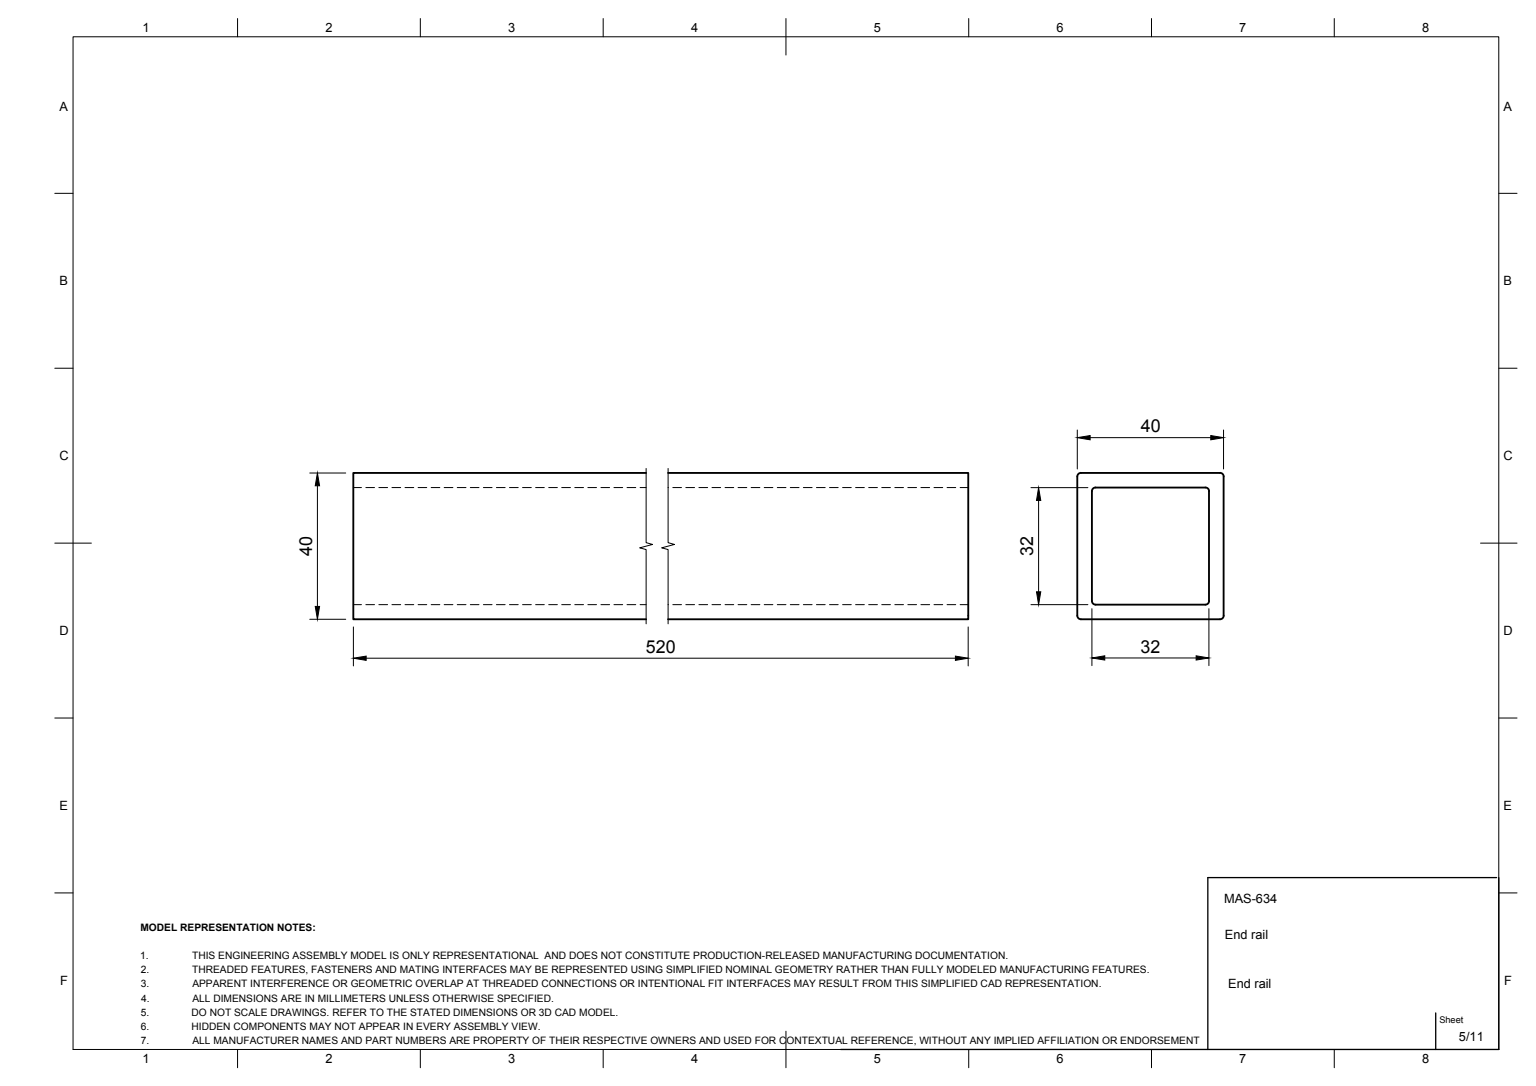
ISO-10303-21;
HEADER;
/* Generated by software containing ST-Developer
 * from STEP Tools, Inc. (www.steptools.com) 
 */

FILE_DESCRIPTION(
/* description */ ('Independent AHU equipment rack. Nominal800x600 frame on1000long40squa
re aluminum posts; two removable notched shelves; welded perimeter/cro
ss rails and rear gussets; two mounting channels; four isolation pads 
and anchor-ready feet. Imported native extrusion library retained and 
cut-length parameters customized per family. Shelf hardware uses model
ed M6 rivet nuts and screws. Weld design, floor anchors and load ratin
g require engineering selection.'),
/* implementation_level */ '2;1');

FILE_NAME(
/* name */ 'End rail.step',
/* time_stamp */ '2026-11-07T19:04:45-08:00',
/* author */ (''),
/* organization */ (''),
/* preprocessor_version */ 'ST-DEVELOPER v20.2',
/* originating_system */ 'Autodesk Translation Framework v15.17.0.0',
/* authorisation */ '');

FILE_SCHEMA (('AUTOMOTIVE_DESIGN { 1 0 10303 214 3 1 1 }'));
ENDSEC;

DATA;
#10=MECHANICAL_DESIGN_GEOMETRIC_PRESENTATION_REPRESENTATION('',(#337),#9777);
#315=SHAPE_REPRESENTATION_RELATIONSHIP('SRR','None',#9859,#326);
#326=ADVANCED_BREP_SHAPE_REPRESENTATION('',(#348),#9768);
#337=STYLED_ITEM('',(#9922),#348);
#348=MANIFOLD_SOLID_BREP('Aluminum square hollow profile',#3842);
#365=FACE_BOUND('',#749,.T.);
#366=FACE_BOUND('',#765,.T.);
#430=PLANE('',#4054);
#431=PLANE('',#4055);
#432=PLANE('',#4065);
#433=PLANE('',#4072);
#434=PLANE('',#4075);
#435=PLANE('',#4078);
#436=PLANE('',#4081);
#437=PLANE('',#4082);
#438=PLANE('',#4083);
#439=PLANE('',#4084);
#540=FACE_OUTER_BOUND('',#746,.T.);
#541=FACE_OUTER_BOUND('',#747,.T.);
#542=FACE_OUTER_BOUND('',#748,.T.);
#543=FACE_OUTER_BOUND('',#750,.T.);
#544=FACE_OUTER_BOUND('',#751,.T.);
#545=FACE_OUTER_BOUND('',#752,.T.);
#546=FACE_OUTER_BOUND('',#753,.T.);
#547=FACE_OUTER_BOUND('',#754,.T.);
#548=FACE_OUTER_BOUND('',#755,.T.);
#549=FACE_OUTER_BOUND('',#756,.T.);
#550=FACE_OUTER_BOUND('',#757,.T.);
#551=FACE_OUTER_BOUND('',#758,.T.);
#552=FACE_OUTER_BOUND('',#759,.T.);
#553=FACE_OUTER_BOUND('',#760,.T.);
#554=FACE_OUTER_BOUND('',#761,.T.);
#555=FACE_OUTER_BOUND('',#762,.T.);
#556=FACE_OUTER_BOUND('',#763,.T.);
#557=FACE_OUTER_BOUND('',#764,.T.);
#746=EDGE_LOOP('',(#2719,#2720,#2721,#2722));
#747=EDGE_LOOP('',(#2723,#2724,#2725,#2726));
#748=EDGE_LOOP('',(#2727,#2728,#2729,#2730,#2731,#2732,#2733,#2734));
#749=EDGE_LOOP('',(#2735,#2736,#2737,#2738,#2739,#2740,#2741,#2742));
#750=EDGE_LOOP('',(#2743,#2744,#2745,#2746));
#751=EDGE_LOOP('',(#2747,#2748,#2749,#2750));
#752=EDGE_LOOP('',(#2751,#2752,#2753,#2754));
#753=EDGE_LOOP('',(#2755,#2756,#2757,#2758));
#754=EDGE_LOOP('',(#2759,#2760,#2761,#2762));
#755=EDGE_LOOP('',(#2763,#2764,#2765,#2766));
#756=EDGE_LOOP('',(#2767,#2768,#2769,#2770));
#757=EDGE_LOOP('',(#2771,#2772,#2773,#2774));
#758=EDGE_LOOP('',(#2775,#2776,#2777,#2778));
#759=EDGE_LOOP('',(#2779,#2780,#2781,#2782));
#760=EDGE_LOOP('',(#2783,#2784,#2785,#2786));
#761=EDGE_LOOP('',(#2787,#2788,#2789,#2790));
#762=EDGE_LOOP('',(#2791,#2792,#2793,#2794));
#763=EDGE_LOOP('',(#2795,#2796,#2797,#2798));
#764=EDGE_LOOP('',(#2799,#2800,#2801,#2802,#2803,#2804,#2805,#2806));
#765=EDGE_LOOP('',(#2807,#2808,#2809,#2810,#2811,#2812,#2813,#2814));
#1017=LINE('',#5620,#1310);
#1018=LINE('',#5623,#1311);
#1019=LINE('',#5626,#1312);
#1020=LINE('',#5628,#1313);
#1021=LINE('',#5629,#1314);
#1022=LINE('',#5632,#1315);
#1023=LINE('',#5636,#1316);
#1024=LINE('',#5640,#1317);
#1025=LINE('',#5644,#1318);
#1026=LINE('',#5648,#1319);
#1027=LINE('',#5652,#1320);
#1028=LINE('',#5656,#1321);
#1029=LINE('',#5660,#1322);
#1030=LINE('',#5663,#1323);
#1031=LINE('',#5666,#1324);
#1032=LINE('',#5667,#1325);
#1033=LINE('',#5671,#1326);
#1034=LINE('',#5674,#1327);
#1035=LINE('',#5680,#1328);
#1036=LINE('',#5681,#1329);
#1037=LINE('',#5684,#1330);
#1038=LINE('',#5685,#1331);
#1039=LINE('',#5689,#1332);
#1040=LINE('',#5692,#1333);
#1041=LINE('',#5693,#1334);
#1042=LINE('',#5697,#1335);
#1043=LINE('',#5700,#1336);
#1044=LINE('',#5701,#1337);
#1045=LINE('',#5705,#1338);
#1046=LINE('',#5707,#1339);
#1047=LINE('',#5709,#1340);
#1048=LINE('',#5711,#1341);
#1310=VECTOR('',#4578,10.);
#1311=VECTOR('',#4581,10.);
#1312=VECTOR('',#4584,10.);
#1313=VECTOR('',#4585,10.);
#1314=VECTOR('',#4586,10.);
#1315=VECTOR('',#4589,10.);
#1316=VECTOR('',#4592,10.);
#1317=VECTOR('',#4595,10.);
#1318=VECTOR('',#4598,10.);
#1319=VECTOR('',#4601,10.);
#1320=VECTOR('',#4604,10.);
#1321=VECTOR('',#4607,10.);
#1322=VECTOR('',#4612,10.);
#1323=VECTOR('',#4615,10.);
#1324=VECTOR('',#4618,10.);
#1325=VECTOR('',#4619,10.);
#1326=VECTOR('',#4624,10.);
#1327=VECTOR('',#4627,10.);
#1328=VECTOR('',#4634,10.);
#1329=VECTOR('',#4635,10.);
#1330=VECTOR('',#4638,10.);
#1331=VECTOR('',#4639,10.);
#1332=VECTOR('',#4644,10.);
#1333=VECTOR('',#4647,10.);
#1334=VECTOR('',#4648,10.);
#1335=VECTOR('',#4653,10.);
#1336=VECTOR('',#4656,10.);
#1337=VECTOR('',#4657,10.);
#1338=VECTOR('',#4662,10.);
#1339=VECTOR('',#4665,10.);
#1340=VECTOR('',#4668,10.);
#1341=VECTOR('',#4671,10.);
#1573=CIRCLE('',#4052,1.);
#1574=CIRCLE('',#4053,1.);
#1575=CIRCLE('',#4056,1.);
#1576=CIRCLE('',#4057,1.);
#1577=CIRCLE('',#4058,1.);
#1578=CIRCLE('',#4059,1.);
#1579=CIRCLE('',#4060,1.);
#1580=CIRCLE('',#4061,1.);
#1581=CIRCLE('',#4062,1.);
#1582=CIRCLE('',#4064,1.);
#1583=CIRCLE('',#4067,1.);
#1584=CIRCLE('',#4069,1.);
#1585=CIRCLE('',#4071,1.);
#1586=CIRCLE('',#4074,1.);
#1587=CIRCLE('',#4077,1.);
#1588=CIRCLE('',#4080,1.);
#1728=VERTEX_POINT('',#5616);
#1729=VERTEX_POINT('',#5617);
#1730=VERTEX_POINT('',#5619);
#1731=VERTEX_POINT('',#5621);
#1732=VERTEX_POINT('',#5625);
#1733=VERTEX_POINT('',#5627);
#1734=VERTEX_POINT('',#5631);
#1735=VERTEX_POINT('',#5633);
#1736=VERTEX_POINT('',#5635);
#1737=VERTEX_POINT('',#5637);
#1738=VERTEX_POINT('',#5639);
#1739=VERTEX_POINT('',#5642);
#1740=VERTEX_POINT('',#5643);
#1741=VERTEX_POINT('',#5645);
#1742=VERTEX_POINT('',#5647);
#1743=VERTEX_POINT('',#5649);
#1744=VERTEX_POINT('',#5651);
#1745=VERTEX_POINT('',#5653);
#1746=VERTEX_POINT('',#5655);
#1747=VERTEX_POINT('',#5659);
#1748=VERTEX_POINT('',#5661);
#1749=VERTEX_POINT('',#5665);
#1750=VERTEX_POINT('',#5669);
#1751=VERTEX_POINT('',#5673);
#1752=VERTEX_POINT('',#5677);
#1753=VERTEX_POINT('',#5678);
#1754=VERTEX_POINT('',#5683);
#1755=VERTEX_POINT('',#5687);
#1756=VERTEX_POINT('',#5691);
#1757=VERTEX_POINT('',#5695);
#1758=VERTEX_POINT('',#5699);
#1759=VERTEX_POINT('',#5703);
#2104=EDGE_CURVE('',#1728,#1729,#1573,.T.);
#2105=EDGE_CURVE('',#1729,#1730,#1017,.T.);
#2106=EDGE_CURVE('',#1730,#1731,#1574,.T.);
#2107=EDGE_CURVE('',#1731,#1728,#1018,.T.);
#2108=EDGE_CURVE('',#1732,#1729,#1019,.T.);
#2109=EDGE_CURVE('',#1733,#1732,#1020,.T.);
#2110=EDGE_CURVE('',#1733,#1730,#1021,.T.);
#2111=EDGE_CURVE('',#1728,#1734,#1022,.T.);
#2112=EDGE_CURVE('',#1735,#1734,#1575,.T.);
#2113=EDGE_CURVE('',#1735,#1736,#1023,.T.);
#2114=EDGE_CURVE('',#1737,#1736,#1576,.T.);
#2115=EDGE_CURVE('',#1737,#1738,#1024,.T.);
#2116=EDGE_CURVE('',#1732,#1738,#1577,.T.);
#2117=EDGE_CURVE('',#1739,#1740,#1025,.T.);
#2118=EDGE_CURVE('',#1741,#1740,#1578,.T.);
#2119=EDGE_CURVE('',#1741,#1742,#1026,.T.);
#2120=EDGE_CURVE('',#1743,#1742,#1579,.T.);
#2121=EDGE_CURVE('',#1743,#1744,#1027,.T.);
#2122=EDGE_CURVE('',#1745,#1744,#1580,.T.);
#2123=EDGE_CURVE('',#1745,#1746,#1028,.T.);
#2124=EDGE_CURVE('',#1739,#1746,#1581,.T.);
#2125=EDGE_CURVE('',#1734,#1747,#1029,.T.);
#2126=EDGE_CURVE('',#1747,#1748,#1582,.T.);
#2127=EDGE_CURVE('',#1748,#1735,#1030,.T.);
#2128=EDGE_CURVE('',#1748,#1749,#1031,.T.);
#2129=EDGE_CURVE('',#1736,#1749,#1032,.T.);
#2130=EDGE_CURVE('',#1749,#1750,#1583,.T.);
#2131=EDGE_CURVE('',#1750,#1737,#1033,.T.);
#2132=EDGE_CURVE('',#1738,#1751,#1034,.T.);
#2133=EDGE_CURVE('',#1751,#1733,#1584,.T.);
#2134=EDGE_CURVE('',#1752,#1753,#1585,.T.);
#2135=EDGE_CURVE('',#1753,#1741,#1035,.T.);
#2136=EDGE_CURVE('',#1740,#1752,#1036,.T.);
#2137=EDGE_CURVE('',#1753,#1754,#1037,.T.);
#2138=EDGE_CURVE('',#1742,#1754,#1038,.T.);
#2139=EDGE_CURVE('',#1754,#1755,#1586,.T.);
#2140=EDGE_CURVE('',#1755,#1743,#1039,.T.);
#2141=EDGE_CURVE('',#1755,#1756,#1040,.T.);
#2142=EDGE_CURVE('',#1744,#1756,#1041,.T.);
#2143=EDGE_CURVE('',#1756,#1757,#1587,.T.);
#2144=EDGE_CURVE('',#1757,#1745,#1042,.T.);
#2145=EDGE_CURVE('',#1757,#1758,#1043,.T.);
#2146=EDGE_CURVE('',#1746,#1758,#1044,.T.);
#2147=EDGE_CURVE('',#1758,#1759,#1588,.T.);
#2148=EDGE_CURVE('',#1759,#1739,#1045,.T.);
#2149=EDGE_CURVE('',#1759,#1752,#1046,.T.);
#2150=EDGE_CURVE('',#1750,#1751,#1047,.T.);
#2151=EDGE_CURVE('',#1731,#1747,#1048,.T.);
#2719=ORIENTED_EDGE('',*,*,#2104,.T.);
#2720=ORIENTED_EDGE('',*,*,#2105,.T.);
#2721=ORIENTED_EDGE('',*,*,#2106,.T.);
#2722=ORIENTED_EDGE('',*,*,#2107,.T.);
#2723=ORIENTED_EDGE('',*,*,#2105,.F.);
#2724=ORIENTED_EDGE('',*,*,#2108,.F.);
#2725=ORIENTED_EDGE('',*,*,#2109,.F.);
#2726=ORIENTED_EDGE('',*,*,#2110,.T.);
#2727=ORIENTED_EDGE('',*,*,#2104,.F.);
#2728=ORIENTED_EDGE('',*,*,#2111,.T.);
#2729=ORIENTED_EDGE('',*,*,#2112,.F.);
#2730=ORIENTED_EDGE('',*,*,#2113,.T.);
#2731=ORIENTED_EDGE('',*,*,#2114,.F.);
#2732=ORIENTED_EDGE('',*,*,#2115,.T.);
#2733=ORIENTED_EDGE('',*,*,#2116,.F.);
#2734=ORIENTED_EDGE('',*,*,#2108,.T.);
#2735=ORIENTED_EDGE('',*,*,#2117,.T.);
#2736=ORIENTED_EDGE('',*,*,#2118,.F.);
#2737=ORIENTED_EDGE('',*,*,#2119,.T.);
#2738=ORIENTED_EDGE('',*,*,#2120,.F.);
#2739=ORIENTED_EDGE('',*,*,#2121,.T.);
#2740=ORIENTED_EDGE('',*,*,#2122,.F.);
#2741=ORIENTED_EDGE('',*,*,#2123,.T.);
#2742=ORIENTED_EDGE('',*,*,#2124,.F.);
#2743=ORIENTED_EDGE('',*,*,#2112,.T.);
#2744=ORIENTED_EDGE('',*,*,#2125,.T.);
#2745=ORIENTED_EDGE('',*,*,#2126,.T.);
#2746=ORIENTED_EDGE('',*,*,#2127,.T.);
#2747=ORIENTED_EDGE('',*,*,#2127,.F.);
#2748=ORIENTED_EDGE('',*,*,#2128,.T.);
#2749=ORIENTED_EDGE('',*,*,#2129,.F.);
#2750=ORIENTED_EDGE('',*,*,#2113,.F.);
#2751=ORIENTED_EDGE('',*,*,#2114,.T.);
#2752=ORIENTED_EDGE('',*,*,#2129,.T.);
#2753=ORIENTED_EDGE('',*,*,#2130,.T.);
#2754=ORIENTED_EDGE('',*,*,#2131,.T.);
#2755=ORIENTED_EDGE('',*,*,#2116,.T.);
#2756=ORIENTED_EDGE('',*,*,#2132,.T.);
#2757=ORIENTED_EDGE('',*,*,#2133,.T.);
#2758=ORIENTED_EDGE('',*,*,#2109,.T.);
#2759=ORIENTED_EDGE('',*,*,#2134,.T.);
#2760=ORIENTED_EDGE('',*,*,#2135,.T.);
#2761=ORIENTED_EDGE('',*,*,#2118,.T.);
#2762=ORIENTED_EDGE('',*,*,#2136,.T.);
#2763=ORIENTED_EDGE('',*,*,#2135,.F.);
#2764=ORIENTED_EDGE('',*,*,#2137,.T.);
#2765=ORIENTED_EDGE('',*,*,#2138,.F.);
#2766=ORIENTED_EDGE('',*,*,#2119,.F.);
#2767=ORIENTED_EDGE('',*,*,#2139,.T.);
#2768=ORIENTED_EDGE('',*,*,#2140,.T.);
#2769=ORIENTED_EDGE('',*,*,#2120,.T.);
#2770=ORIENTED_EDGE('',*,*,#2138,.T.);
#2771=ORIENTED_EDGE('',*,*,#2140,.F.);
#2772=ORIENTED_EDGE('',*,*,#2141,.T.);
#2773=ORIENTED_EDGE('',*,*,#2142,.F.);
#2774=ORIENTED_EDGE('',*,*,#2121,.F.);
#2775=ORIENTED_EDGE('',*,*,#2143,.T.);
#2776=ORIENTED_EDGE('',*,*,#2144,.T.);
#2777=ORIENTED_EDGE('',*,*,#2122,.T.);
#2778=ORIENTED_EDGE('',*,*,#2142,.T.);
#2779=ORIENTED_EDGE('',*,*,#2144,.F.);
#2780=ORIENTED_EDGE('',*,*,#2145,.T.);
#2781=ORIENTED_EDGE('',*,*,#2146,.F.);
#2782=ORIENTED_EDGE('',*,*,#2123,.F.);
#2783=ORIENTED_EDGE('',*,*,#2147,.T.);
#2784=ORIENTED_EDGE('',*,*,#2148,.T.);
#2785=ORIENTED_EDGE('',*,*,#2124,.T.);
#2786=ORIENTED_EDGE('',*,*,#2146,.T.);
#2787=ORIENTED_EDGE('',*,*,#2136,.F.);
#2788=ORIENTED_EDGE('',*,*,#2117,.F.);
#2789=ORIENTED_EDGE('',*,*,#2148,.F.);
#2790=ORIENTED_EDGE('',*,*,#2149,.T.);
#2791=ORIENTED_EDGE('',*,*,#2131,.F.);
#2792=ORIENTED_EDGE('',*,*,#2150,.T.);
#2793=ORIENTED_EDGE('',*,*,#2132,.F.);
#2794=ORIENTED_EDGE('',*,*,#2115,.F.);
#2795=ORIENTED_EDGE('',*,*,#2107,.F.);
#2796=ORIENTED_EDGE('',*,*,#2151,.T.);
#2797=ORIENTED_EDGE('',*,*,#2125,.F.);
#2798=ORIENTED_EDGE('',*,*,#2111,.F.);
#2799=ORIENTED_EDGE('',*,*,#2106,.F.);
#2800=ORIENTED_EDGE('',*,*,#2110,.F.);
#2801=ORIENTED_EDGE('',*,*,#2133,.F.);
#2802=ORIENTED_EDGE('',*,*,#2150,.F.);
#2803=ORIENTED_EDGE('',*,*,#2130,.F.);
#2804=ORIENTED_EDGE('',*,*,#2128,.F.);
#2805=ORIENTED_EDGE('',*,*,#2126,.F.);
#2806=ORIENTED_EDGE('',*,*,#2151,.F.);
#2807=ORIENTED_EDGE('',*,*,#2147,.F.);
#2808=ORIENTED_EDGE('',*,*,#2145,.F.);
#2809=ORIENTED_EDGE('',*,*,#2143,.F.);
#2810=ORIENTED_EDGE('',*,*,#2141,.F.);
#2811=ORIENTED_EDGE('',*,*,#2139,.F.);
#2812=ORIENTED_EDGE('',*,*,#2137,.F.);
#2813=ORIENTED_EDGE('',*,*,#2134,.F.);
#2814=ORIENTED_EDGE('',*,*,#2149,.F.);
#3559=CYLINDRICAL_SURFACE('',#4051,1.);
#3560=CYLINDRICAL_SURFACE('',#4063,1.);
#3561=CYLINDRICAL_SURFACE('',#4066,1.);
#3562=CYLINDRICAL_SURFACE('',#4068,1.);
#3563=CYLINDRICAL_SURFACE('',#4070,1.);
#3564=CYLINDRICAL_SURFACE('',#4073,1.);
#3565=CYLINDRICAL_SURFACE('',#4076,1.);
#3566=CYLINDRICAL_SURFACE('',#4079,1.);
#3680=ADVANCED_FACE('',(#540),#3559,.T.);
#3681=ADVANCED_FACE('',(#541),#430,.T.);
#3682=ADVANCED_FACE('',(#542,#365),#431,.T.);
#3683=ADVANCED_FACE('',(#543),#3560,.T.);
#3684=ADVANCED_FACE('',(#544),#432,.T.);
#3685=ADVANCED_FACE('',(#545),#3561,.T.);
#3686=ADVANCED_FACE('',(#546),#3562,.T.);
#3687=ADVANCED_FACE('',(#547),#3563,.F.);
#3688=ADVANCED_FACE('',(#548),#433,.T.);
#3689=ADVANCED_FACE('',(#549),#3564,.F.);
#3690=ADVANCED_FACE('',(#550),#434,.T.);
#3691=ADVANCED_FACE('',(#551),#3565,.F.);
#3692=ADVANCED_FACE('',(#552),#435,.T.);
#3693=ADVANCED_FACE('',(#553),#3566,.F.);
#3694=ADVANCED_FACE('',(#554),#436,.T.);
#3695=ADVANCED_FACE('',(#555),#437,.T.);
#3696=ADVANCED_FACE('',(#556),#438,.T.);
#3697=ADVANCED_FACE('',(#557,#366),#439,.F.);
#3842=CLOSED_SHELL('',(#3680,#3681,#3682,#3683,#3684,#3685,#3686,#3687,
#3688,#3689,#3690,#3691,#3692,#3693,#3694,#3695,#3696,#3697));
#4050=AXIS2_PLACEMENT_3D('',#5614,#4572,#4573);
#4051=AXIS2_PLACEMENT_3D('',#5615,#4574,#4575);
#4052=AXIS2_PLACEMENT_3D('',#5618,#4576,#4577);
#4053=AXIS2_PLACEMENT_3D('',#5622,#4579,#4580);
#4054=AXIS2_PLACEMENT_3D('',#5624,#4582,#4583);
#4055=AXIS2_PLACEMENT_3D('',#5630,#4587,#4588);
#4056=AXIS2_PLACEMENT_3D('',#5634,#4590,#4591);
#4057=AXIS2_PLACEMENT_3D('',#5638,#4593,#4594);
#4058=AXIS2_PLACEMENT_3D('',#5641,#4596,#4597);
#4059=AXIS2_PLACEMENT_3D('',#5646,#4599,#4600);
#4060=AXIS2_PLACEMENT_3D('',#5650,#4602,#4603);
#4061=AXIS2_PLACEMENT_3D('',#5654,#4605,#4606);
#4062=AXIS2_PLACEMENT_3D('',#5657,#4608,#4609);
#4063=AXIS2_PLACEMENT_3D('',#5658,#4610,#4611);
#4064=AXIS2_PLACEMENT_3D('',#5662,#4613,#4614);
#4065=AXIS2_PLACEMENT_3D('',#5664,#4616,#4617);
#4066=AXIS2_PLACEMENT_3D('',#5668,#4620,#4621);
#4067=AXIS2_PLACEMENT_3D('',#5670,#4622,#4623);
#4068=AXIS2_PLACEMENT_3D('',#5672,#4625,#4626);
#4069=AXIS2_PLACEMENT_3D('',#5675,#4628,#4629);
#4070=AXIS2_PLACEMENT_3D('',#5676,#4630,#4631);
#4071=AXIS2_PLACEMENT_3D('',#5679,#4632,#4633);
#4072=AXIS2_PLACEMENT_3D('',#5682,#4636,#4637);
#4073=AXIS2_PLACEMENT_3D('',#5686,#4640,#4641);
#4074=AXIS2_PLACEMENT_3D('',#5688,#4642,#4643);
#4075=AXIS2_PLACEMENT_3D('',#5690,#4645,#4646);
#4076=AXIS2_PLACEMENT_3D('',#5694,#4649,#4650);
#4077=AXIS2_PLACEMENT_3D('',#5696,#4651,#4652);
#4078=AXIS2_PLACEMENT_3D('',#5698,#4654,#4655);
#4079=AXIS2_PLACEMENT_3D('',#5702,#4658,#4659);
#4080=AXIS2_PLACEMENT_3D('',#5704,#4660,#4661);
#4081=AXIS2_PLACEMENT_3D('',#5706,#4663,#4664);
#4082=AXIS2_PLACEMENT_3D('',#5708,#4666,#4667);
#4083=AXIS2_PLACEMENT_3D('',#5710,#4669,#4670);
#4084=AXIS2_PLACEMENT_3D('',#5712,#4672,#4673);
#4572=DIRECTION('axis',(0.,0.,1.));
#4573=DIRECTION('refdir',(1.,0.,0.));
#4574=DIRECTION('center_axis',(0.,0.,1.));
#4575=DIRECTION('ref_axis',(-0.707106781186548,-0.707106781186548,0.));
#4576=DIRECTION('center_axis',(0.,0.,-1.));
#4577=DIRECTION('ref_axis',(-0.707106781186548,-0.707106781186548,0.));
#4578=DIRECTION('',(0.,0.,-1.));
#4579=DIRECTION('center_axis',(0.,0.,1.));
#4580=DIRECTION('ref_axis',(-0.707106781186548,-0.707106781186548,0.));
#4581=DIRECTION('',(0.,0.,1.));
#4582=DIRECTION('center_axis',(-1.,0.,0.));
#4583=DIRECTION('ref_axis',(0.,-1.,0.));
#4584=DIRECTION('',(0.,-1.,0.));
#4585=DIRECTION('',(0.,0.,1.));
#4586=DIRECTION('',(0.,-1.,0.));
#4587=DIRECTION('center_axis',(0.,0.,1.));
#4588=DIRECTION('ref_axis',(1.,0.,0.));
#4589=DIRECTION('',(1.,0.,0.));
#4590=DIRECTION('center_axis',(0.,0.,-1.));
#4591=DIRECTION('ref_axis',(0.707106781186548,-0.707106781186548,0.));
#4592=DIRECTION('',(0.,1.,0.));
#4593=DIRECTION('center_axis',(0.,0.,-1.));
#4594=DIRECTION('ref_axis',(0.707106781186548,0.707106781186548,0.));
#4595=DIRECTION('',(-1.,0.,0.));
#4596=DIRECTION('center_axis',(0.,0.,-1.));
#4597=DIRECTION('ref_axis',(-0.707106781186548,0.707106781186548,0.));
#4598=DIRECTION('',(0.,1.,0.));
#4599=DIRECTION('center_axis',(0.,0.,1.));
#4600=DIRECTION('ref_axis',(-0.707106781186548,0.707106781186548,0.));
#4601=DIRECTION('',(1.,0.,0.));
#4602=DIRECTION('center_axis',(0.,0.,1.));
#4603=DIRECTION('ref_axis',(0.707106781186548,0.707106781186548,0.));
#4604=DIRECTION('',(0.,-1.,0.));
#4605=DIRECTION('center_axis',(0.,0.,1.));
#4606=DIRECTION('ref_axis',(0.707106781186548,-0.707106781186548,0.));
#4607=DIRECTION('',(-1.,0.,0.));
#4608=DIRECTION('center_axis',(0.,0.,1.));
#4609=DIRECTION('ref_axis',(-0.707106781186548,-0.707106781186548,0.));
#4610=DIRECTION('center_axis',(0.,0.,1.));
#4611=DIRECTION('ref_axis',(0.707106781186548,-0.707106781186548,0.));
#4612=DIRECTION('',(0.,0.,-1.));
#4613=DIRECTION('center_axis',(0.,0.,1.));
#4614=DIRECTION('ref_axis',(0.707106781186548,-0.707106781186548,0.));
#4615=DIRECTION('',(0.,0.,1.));
#4616=DIRECTION('center_axis',(1.,0.,0.));
#4617=DIRECTION('ref_axis',(0.,1.,0.));
#4618=DIRECTION('',(0.,1.,0.));
#4619=DIRECTION('',(0.,0.,-1.));
#4620=DIRECTION('center_axis',(0.,0.,1.));
#4621=DIRECTION('ref_axis',(0.707106781186548,0.707106781186548,0.));
#4622=DIRECTION('center_axis',(0.,0.,1.));
#4623=DIRECTION('ref_axis',(0.707106781186548,0.707106781186548,0.));
#4624=DIRECTION('',(0.,0.,1.));
#4625=DIRECTION('center_axis',(0.,0.,1.));
#4626=DIRECTION('ref_axis',(-0.707106781186548,0.707106781186548,0.));
#4627=DIRECTION('',(0.,0.,-1.));
#4628=DIRECTION('center_axis',(0.,0.,1.));
#4629=DIRECTION('ref_axis',(-0.707106781186548,0.707106781186548,0.));
#4630=DIRECTION('center_axis',(0.,0.,1.));
#4631=DIRECTION('ref_axis',(-0.707106781186548,0.707106781186548,0.));
#4632=DIRECTION('center_axis',(0.,0.,-1.));
#4633=DIRECTION('ref_axis',(-0.707106781186548,0.707106781186548,0.));
#4634=DIRECTION('',(0.,0.,1.));
#4635=DIRECTION('',(0.,0.,-1.));
#4636=DIRECTION('center_axis',(0.,-1.,0.));
#4637=DIRECTION('ref_axis',(1.,0.,0.));
#4638=DIRECTION('',(1.,0.,0.));
#4639=DIRECTION('',(0.,0.,-1.));
#4640=DIRECTION('center_axis',(0.,0.,1.));
#4641=DIRECTION('ref_axis',(0.707106781186548,0.707106781186548,0.));
#4642=DIRECTION('center_axis',(0.,0.,-1.));
#4643=DIRECTION('ref_axis',(0.707106781186548,0.707106781186548,0.));
#4644=DIRECTION('',(0.,0.,1.));
#4645=DIRECTION('center_axis',(-1.,0.,0.));
#4646=DIRECTION('ref_axis',(0.,-1.,0.));
#4647=DIRECTION('',(0.,-1.,0.));
#4648=DIRECTION('',(0.,0.,-1.));
#4649=DIRECTION('center_axis',(0.,0.,1.));
#4650=DIRECTION('ref_axis',(0.707106781186548,-0.707106781186548,0.));
#4651=DIRECTION('center_axis',(0.,0.,-1.));
#4652=DIRECTION('ref_axis',(0.707106781186548,-0.707106781186548,0.));
#4653=DIRECTION('',(0.,0.,1.));
#4654=DIRECTION('center_axis',(0.,1.,0.));
#4655=DIRECTION('ref_axis',(-1.,0.,0.));
#4656=DIRECTION('',(-1.,0.,0.));
#4657=DIRECTION('',(0.,0.,-1.));
#4658=DIRECTION('center_axis',(0.,0.,1.));
#4659=DIRECTION('ref_axis',(-0.707106781186548,-0.707106781186548,0.));
#4660=DIRECTION('center_axis',(0.,0.,-1.));
#4661=DIRECTION('ref_axis',(-0.707106781186548,-0.707106781186548,0.));
#4662=DIRECTION('',(0.,0.,1.));
#4663=DIRECTION('center_axis',(1.,0.,0.));
#4664=DIRECTION('ref_axis',(0.,1.,0.));
#4665=DIRECTION('',(0.,1.,0.));
#4666=DIRECTION('center_axis',(0.,1.,0.));
#4667=DIRECTION('ref_axis',(-1.,0.,0.));
#4668=DIRECTION('',(-1.,0.,0.));
#4669=DIRECTION('center_axis',(0.,-1.,0.));
#4670=DIRECTION('ref_axis',(1.,0.,0.));
#4671=DIRECTION('',(1.,0.,0.));
#4672=DIRECTION('center_axis',(0.,0.,1.));
#4673=DIRECTION('ref_axis',(1.,0.,0.));
#5614=CARTESIAN_POINT('',(0.,0.,0.));
#5615=CARTESIAN_POINT('Origin',(-19.,-19.,0.));
#5616=CARTESIAN_POINT('',(-19.,-20.,520.));
#5617=CARTESIAN_POINT('',(-20.,-19.,520.));
#5618=CARTESIAN_POINT('Origin',(-19.,-19.,520.));
#5619=CARTESIAN_POINT('',(-20.,-19.,0.));
#5620=CARTESIAN_POINT('',(-20.,-19.,0.));
#5621=CARTESIAN_POINT('',(-19.,-20.,0.));
#5622=CARTESIAN_POINT('Origin',(-19.,-19.,0.));
#5623=CARTESIAN_POINT('',(-19.,-20.,0.));
#5624=CARTESIAN_POINT('Origin',(-20.,20.,0.));
#5625=CARTESIAN_POINT('',(-20.,19.,520.));
#5626=CARTESIAN_POINT('',(-20.,20.,520.));
#5627=CARTESIAN_POINT('',(-20.,19.,0.));
#5628=CARTESIAN_POINT('',(-20.,19.,0.));
#5629=CARTESIAN_POINT('',(-20.,20.,0.));
#5630=CARTESIAN_POINT('Origin',(0.,0.,520.));
#5631=CARTESIAN_POINT('',(19.,-20.,520.));
#5632=CARTESIAN_POINT('',(-20.,-20.,520.));
#5633=CARTESIAN_POINT('',(20.,-19.,520.));
#5634=CARTESIAN_POINT('Origin',(19.,-19.,520.));
#5635=CARTESIAN_POINT('',(20.,19.,520.));
#5636=CARTESIAN_POINT('',(20.,-20.,520.));
#5637=CARTESIAN_POINT('',(19.,20.,520.));
#5638=CARTESIAN_POINT('Origin',(19.,19.,520.));
#5639=CARTESIAN_POINT('',(-19.,20.,520.));
#5640=CARTESIAN_POINT('',(20.,20.,520.));
#5641=CARTESIAN_POINT('Origin',(-19.,19.,520.));
#5642=CARTESIAN_POINT('',(-16.,-15.,520.));
#5643=CARTESIAN_POINT('',(-16.,15.,520.));
#5644=CARTESIAN_POINT('',(-16.,16.,520.));
#5645=CARTESIAN_POINT('',(-15.,16.,520.));
#5646=CARTESIAN_POINT('Origin',(-15.,15.,520.));
#5647=CARTESIAN_POINT('',(15.,16.,520.));
#5648=CARTESIAN_POINT('',(16.,16.,520.));
#5649=CARTESIAN_POINT('',(16.,15.,520.));
#5650=CARTESIAN_POINT('Origin',(15.,15.,520.));
#5651=CARTESIAN_POINT('',(16.,-15.,520.));
#5652=CARTESIAN_POINT('',(16.,-16.,520.));
#5653=CARTESIAN_POINT('',(15.,-16.,520.));
#5654=CARTESIAN_POINT('Origin',(15.,-15.,520.));
#5655=CARTESIAN_POINT('',(-15.,-16.,520.));
#5656=CARTESIAN_POINT('',(-16.,-16.,520.));
#5657=CARTESIAN_POINT('Origin',(-15.,-15.,520.));
#5658=CARTESIAN_POINT('Origin',(19.,-19.,0.));
#5659=CARTESIAN_POINT('',(19.,-20.,0.));
#5660=CARTESIAN_POINT('',(19.,-20.,0.));
#5661=CARTESIAN_POINT('',(20.,-19.,0.));
#5662=CARTESIAN_POINT('Origin',(19.,-19.,0.));
#5663=CARTESIAN_POINT('',(20.,-19.,0.));
#5664=CARTESIAN_POINT('Origin',(20.,-20.,0.));
#5665=CARTESIAN_POINT('',(20.,19.,0.));
#5666=CARTESIAN_POINT('',(20.,-20.,0.));
#5667=CARTESIAN_POINT('',(20.,19.,0.));
#5668=CARTESIAN_POINT('Origin',(19.,19.,0.));
#5669=CARTESIAN_POINT('',(19.,20.,0.));
#5670=CARTESIAN_POINT('Origin',(19.,19.,0.));
#5671=CARTESIAN_POINT('',(19.,20.,0.));
#5672=CARTESIAN_POINT('Origin',(-19.,19.,0.));
#5673=CARTESIAN_POINT('',(-19.,20.,0.));
#5674=CARTESIAN_POINT('',(-19.,20.,0.));
#5675=CARTESIAN_POINT('Origin',(-19.,19.,0.));
#5676=CARTESIAN_POINT('Origin',(-15.,15.,0.));
#5677=CARTESIAN_POINT('',(-16.,15.,0.));
#5678=CARTESIAN_POINT('',(-15.,16.,0.));
#5679=CARTESIAN_POINT('Origin',(-15.,15.,0.));
#5680=CARTESIAN_POINT('',(-15.,16.,0.));
#5681=CARTESIAN_POINT('',(-16.,15.,0.));
#5682=CARTESIAN_POINT('Origin',(-16.,16.,0.));
#5683=CARTESIAN_POINT('',(15.,16.,0.));
#5684=CARTESIAN_POINT('',(16.,16.,0.));
#5685=CARTESIAN_POINT('',(15.,16.,0.));
#5686=CARTESIAN_POINT('Origin',(15.,15.,0.));
#5687=CARTESIAN_POINT('',(16.,15.,0.));
#5688=CARTESIAN_POINT('Origin',(15.,15.,0.));
#5689=CARTESIAN_POINT('',(16.,15.,0.));
#5690=CARTESIAN_POINT('Origin',(16.,16.,0.));
#5691=CARTESIAN_POINT('',(16.,-15.,0.));
#5692=CARTESIAN_POINT('',(16.,-16.,0.));
#5693=CARTESIAN_POINT('',(16.,-15.,0.));
#5694=CARTESIAN_POINT('Origin',(15.,-15.,0.));
#5695=CARTESIAN_POINT('',(15.,-16.,0.));
#5696=CARTESIAN_POINT('Origin',(15.,-15.,0.));
#5697=CARTESIAN_POINT('',(15.,-16.,0.));
#5698=CARTESIAN_POINT('Origin',(16.,-16.,0.));
#5699=CARTESIAN_POINT('',(-15.,-16.,0.));
#5700=CARTESIAN_POINT('',(-16.,-16.,0.));
#5701=CARTESIAN_POINT('',(-15.,-16.,0.));
#5702=CARTESIAN_POINT('Origin',(-15.,-15.,0.));
#5703=CARTESIAN_POINT('',(-16.,-15.,0.));
#5704=CARTESIAN_POINT('Origin',(-15.,-15.,0.));
#5705=CARTESIAN_POINT('',(-16.,-15.,0.));
#5706=CARTESIAN_POINT('Origin',(-16.,-16.,0.));
#5707=CARTESIAN_POINT('',(-16.,16.,0.));
#5708=CARTESIAN_POINT('Origin',(20.,20.,0.));
#5709=CARTESIAN_POINT('',(20.,20.,0.));
#5710=CARTESIAN_POINT('Origin',(-20.,-20.,0.));
#5711=CARTESIAN_POINT('',(-20.,-20.,0.));
#5712=CARTESIAN_POINT('Origin',(0.,0.,0.));
#9755=UNCERTAINTY_MEASURE_WITH_UNIT(LENGTH_MEASURE(0.01),#9778,
'DISTANCE_ACCURACY_VALUE',
'Maximum model space distance between geometric entities at asserted c
onnectivities');
#9764=UNCERTAINTY_MEASURE_WITH_UNIT(LENGTH_MEASURE(0.01),#9778,
'DISTANCE_ACCURACY_VALUE',
'Maximum model space distance between geometric entities at asserted c
onnectivities');
#9768=(
GEOMETRIC_REPRESENTATION_CONTEXT(3)
GLOBAL_UNCERTAINTY_ASSIGNED_CONTEXT((#9755))
GLOBAL_UNIT_ASSIGNED_CONTEXT((#9778,#9780,#9781))
REPRESENTATION_CONTEXT('','3D')
);
#9777=(
GEOMETRIC_REPRESENTATION_CONTEXT(3)
GLOBAL_UNCERTAINTY_ASSIGNED_CONTEXT((#9764))
GLOBAL_UNIT_ASSIGNED_CONTEXT((#9778,#9780,#9781))
REPRESENTATION_CONTEXT('','3D')
);
#9778=(
LENGTH_UNIT()
NAMED_UNIT(*)
SI_UNIT(.MILLI.,.METRE.)
);
#9780=(
NAMED_UNIT(*)
PLANE_ANGLE_UNIT()
SI_UNIT($,.RADIAN.)
);
#9781=(
NAMED_UNIT(*)
SI_UNIT($,.STERADIAN.)
SOLID_ANGLE_UNIT()
);
#9785=SHAPE_DEFINITION_REPRESENTATION(#9797,#9859);
#9797=PRODUCT_DEFINITION_SHAPE('',$,#9872);
#9859=SHAPE_REPRESENTATION('',(#4050),#9768);
#9868=PRODUCT_DEFINITION_CONTEXT('part definition',#9906,'design');
#9872=PRODUCT_DEFINITION('End rail','End rail',#9884,#9868);
#9884=PRODUCT_DEFINITION_FORMATION('',$,#9911);
#9906=APPLICATION_CONTEXT(
'Core Data for Automotive Mechanical Design Process');
#9907=PRODUCT_CONTEXT('part definition',#9906,'mechanical');
#9911=PRODUCT('End rail','End rail',
'Independent aluminum extrusion section. Whole-mm nominal die dimensio
ns; parametric saw-cut length. Select structural loading, tolerances a
nd finish for the assembly application.',(#9907));
#9922=PRESENTATION_STYLE_ASSIGNMENT((#9933));
#9933=SURFACE_STYLE_USAGE(.BOTH.,#9944);
#9944=SURFACE_SIDE_STYLE('',(#9955));
#9955=SURFACE_STYLE_FILL_AREA(#9966);
#9966=FILL_AREA_STYLE('Dark blue',(#9977));
#9977=FILL_AREA_STYLE_COLOUR('Dark blue',#9988);
#9988=COLOUR_RGB('Dark blue',0.0901960784313725,0.270588235294118,0.513725490196078);
ENDSEC;
END-ISO-10303-21;
